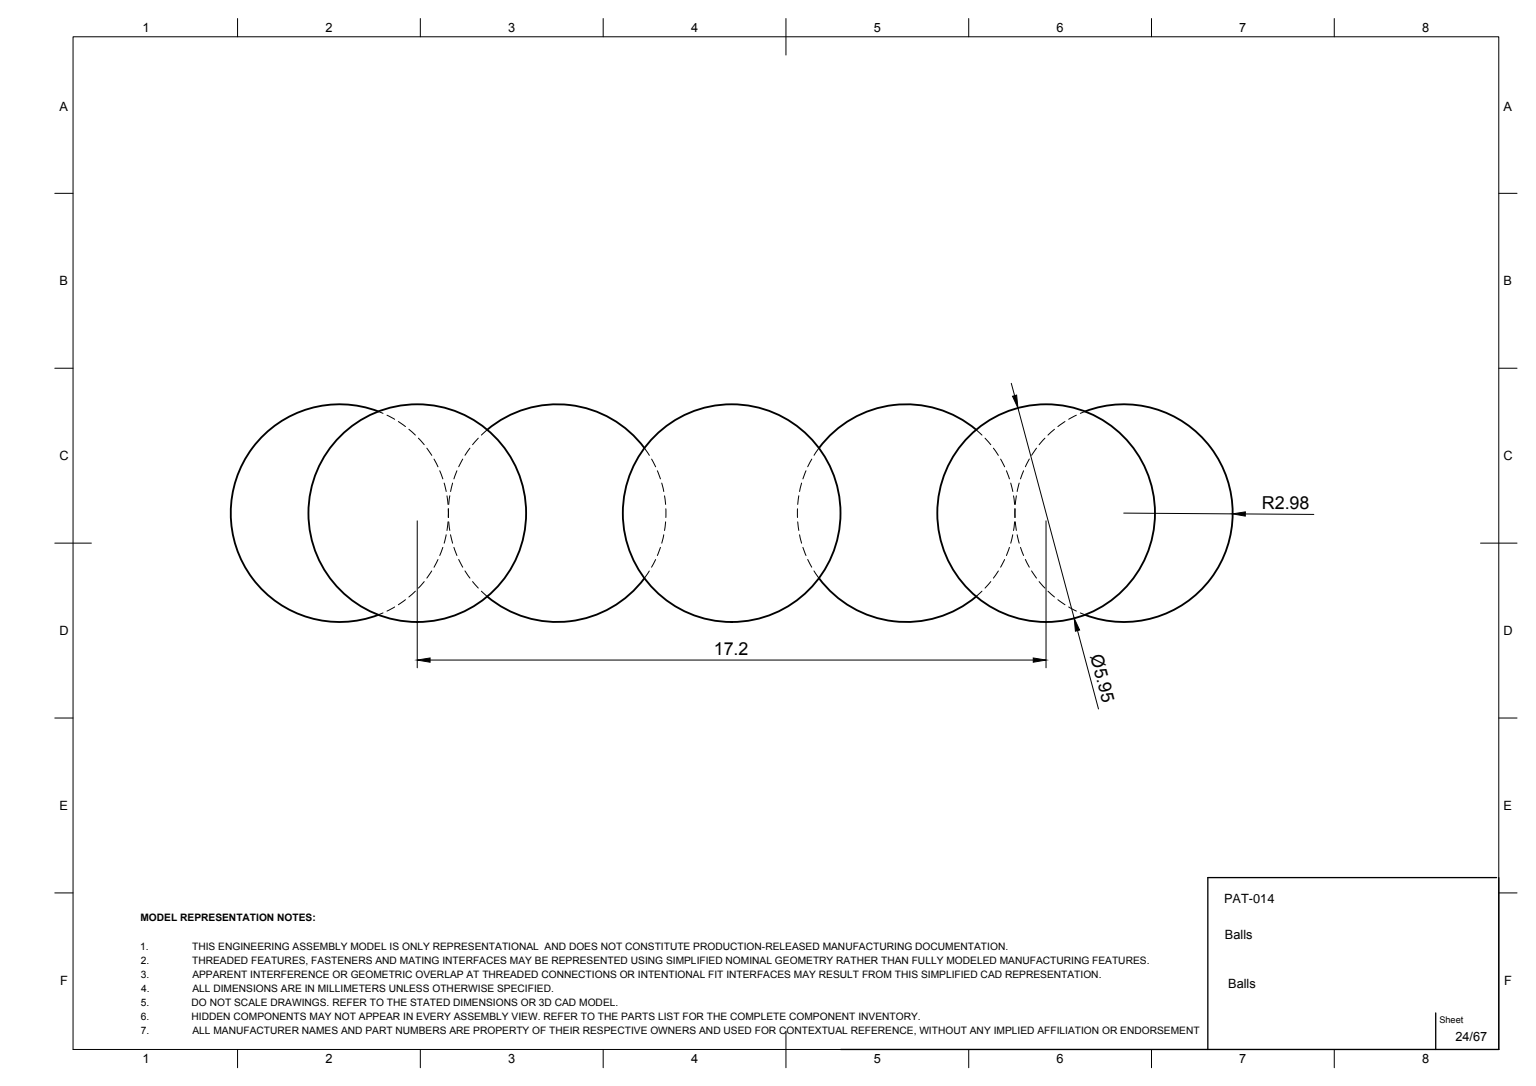
ISO-10303-21;
HEADER;
/* Generated by software containing ST-Developer
 * from STEP Tools, Inc. (www.steptools.com) 
 */

FILE_DESCRIPTION(
/* description */ ('Bin tilter linkage'),
/* implementation_level */ '2;1');

FILE_NAME(
/* name */ 'Balls.step',
/* time_stamp */ '2026-10-28T03:26:24-07:00',
/* author */ (''),
/* organization */ (''),
/* preprocessor_version */ 'ST-DEVELOPER v20.2',
/* originating_system */ 'Autodesk Translation Framework v15.17.0.0',
/* authorisation */ '');

FILE_SCHEMA (('AUTOMOTIVE_DESIGN { 1 0 10303 214 3 1 1 }'));
ENDSEC;

DATA;
#10=MECHANICAL_DESIGN_GEOMETRIC_PRESENTATION_REPRESENTATION('',(#936,#937,#938,#939,#940,#941,#942),#23728);
#613=SPHERICAL_SURFACE('',#14815,0.29765);
#614=SPHERICAL_SURFACE('',#14817,0.29765);
#615=SPHERICAL_SURFACE('',#14819,0.29765);
#616=SPHERICAL_SURFACE('',#14821,0.29765);
#617=SPHERICAL_SURFACE('',#14823,0.29765);
#618=SPHERICAL_SURFACE('',#14825,0.29765);
#619=SPHERICAL_SURFACE('',#14827,0.29765);
#724=SHAPE_REPRESENTATION_RELATIONSHIP('SRR','None',#24191,#830);
#830=ADVANCED_BREP_SHAPE_REPRESENTATION('',(#1049,#1050,#1051,#1052,#1053,
#1054,#1055),#23691);
#936=STYLED_ITEM('',(#24765),#1049);
#937=STYLED_ITEM('',(#24765),#1050);
#938=STYLED_ITEM('',(#24765),#1051);
#939=STYLED_ITEM('',(#24765),#1052);
#940=STYLED_ITEM('',(#24765),#1053);
#941=STYLED_ITEM('',(#24765),#1054);
#942=STYLED_ITEM('',(#24765),#1055);
#1049=MANIFOLD_SOLID_BREP('Body1',#12467);
#1050=MANIFOLD_SOLID_BREP('Body2',#12468);
#1051=MANIFOLD_SOLID_BREP('Body3',#12469);
#1052=MANIFOLD_SOLID_BREP('Body4',#12470);
#1053=MANIFOLD_SOLID_BREP('Body5',#12471);
#1054=MANIFOLD_SOLID_BREP('Body6',#12472);
#1055=MANIFOLD_SOLID_BREP('Body7',#12473);
#2411=FACE_OUTER_BOUND('',#3491,.T.);
#2412=FACE_OUTER_BOUND('',#3492,.T.);
#2413=FACE_OUTER_BOUND('',#3493,.T.);
#2414=FACE_OUTER_BOUND('',#3494,.T.);
#2415=FACE_OUTER_BOUND('',#3495,.T.);
#2416=FACE_OUTER_BOUND('',#3496,.T.);
#2417=FACE_OUTER_BOUND('',#3497,.T.);
#3491=EDGE_LOOP('',(#10277,#10278));
#3492=EDGE_LOOP('',(#10279,#10280));
#3493=EDGE_LOOP('',(#10281,#10282));
#3494=EDGE_LOOP('',(#10283,#10284));
#3495=EDGE_LOOP('',(#10285,#10286));
#3496=EDGE_LOOP('',(#10287,#10288));
#3497=EDGE_LOOP('',(#10289,#10290));
#5737=CIRCLE('',#14816,0.29765);
#5738=CIRCLE('',#14818,0.29765);
#5739=CIRCLE('',#14820,0.29765);
#5740=CIRCLE('',#14822,0.29765);
#5741=CIRCLE('',#14824,0.29765);
#5742=CIRCLE('',#14826,0.29765);
#5743=CIRCLE('',#14828,0.29765);
#6589=VERTEX_POINT('',#21931);
#6590=VERTEX_POINT('',#21932);
#6591=VERTEX_POINT('',#21935);
#6592=VERTEX_POINT('',#21936);
#6593=VERTEX_POINT('',#21939);
#6594=VERTEX_POINT('',#21940);
#6595=VERTEX_POINT('',#21943);
#6596=VERTEX_POINT('',#21944);
#6597=VERTEX_POINT('',#21947);
#6598=VERTEX_POINT('',#21948);
#6599=VERTEX_POINT('',#21951);
#6600=VERTEX_POINT('',#21952);
#6601=VERTEX_POINT('',#21955);
#6602=VERTEX_POINT('',#21956);
#7878=EDGE_CURVE('',#6589,#6590,#5737,.T.);
#7879=EDGE_CURVE('',#6591,#6592,#5738,.T.);
#7880=EDGE_CURVE('',#6593,#6594,#5739,.T.);
#7881=EDGE_CURVE('',#6595,#6596,#5740,.T.);
#7882=EDGE_CURVE('',#6597,#6598,#5741,.T.);
#7883=EDGE_CURVE('',#6599,#6600,#5742,.T.);
#7884=EDGE_CURVE('',#6601,#6602,#5743,.T.);
#10277=ORIENTED_EDGE('',*,*,#7878,.T.);
#10278=ORIENTED_EDGE('',*,*,#7878,.F.);
#10279=ORIENTED_EDGE('',*,*,#7879,.T.);
#10280=ORIENTED_EDGE('',*,*,#7879,.F.);
#10281=ORIENTED_EDGE('',*,*,#7880,.T.);
#10282=ORIENTED_EDGE('',*,*,#7880,.F.);
#10283=ORIENTED_EDGE('',*,*,#7881,.T.);
#10284=ORIENTED_EDGE('',*,*,#7881,.F.);
#10285=ORIENTED_EDGE('',*,*,#7882,.T.);
#10286=ORIENTED_EDGE('',*,*,#7882,.F.);
#10287=ORIENTED_EDGE('',*,*,#7883,.T.);
#10288=ORIENTED_EDGE('',*,*,#7883,.F.);
#10289=ORIENTED_EDGE('',*,*,#7884,.T.);
#10290=ORIENTED_EDGE('',*,*,#7884,.F.);
#12136=ADVANCED_FACE('',(#2411),#613,.T.);
#12137=ADVANCED_FACE('',(#2412),#614,.T.);
#12138=ADVANCED_FACE('',(#2413),#615,.T.);
#12139=ADVANCED_FACE('',(#2414),#616,.T.);
#12140=ADVANCED_FACE('',(#2415),#617,.T.);
#12141=ADVANCED_FACE('',(#2416),#618,.T.);
#12142=ADVANCED_FACE('',(#2417),#619,.T.);
#12467=CLOSED_SHELL('',(#12136));
#12468=CLOSED_SHELL('',(#12137));
#12469=CLOSED_SHELL('',(#12138));
#12470=CLOSED_SHELL('',(#12139));
#12471=CLOSED_SHELL('',(#12140));
#12472=CLOSED_SHELL('',(#12141));
#12473=CLOSED_SHELL('',(#12142));
#14814=AXIS2_PLACEMENT_3D('',#21929,#18164,#18165);
#14815=AXIS2_PLACEMENT_3D('',#21930,#18166,#18167);
#14816=AXIS2_PLACEMENT_3D('',#21933,#18168,#18169);
#14817=AXIS2_PLACEMENT_3D('',#21934,#18170,#18171);
#14818=AXIS2_PLACEMENT_3D('',#21937,#18172,#18173);
#14819=AXIS2_PLACEMENT_3D('',#21938,#18174,#18175);
#14820=AXIS2_PLACEMENT_3D('',#21941,#18176,#18177);
#14821=AXIS2_PLACEMENT_3D('',#21942,#18178,#18179);
#14822=AXIS2_PLACEMENT_3D('',#21945,#18180,#18181);
#14823=AXIS2_PLACEMENT_3D('',#21946,#18182,#18183);
#14824=AXIS2_PLACEMENT_3D('',#21949,#18184,#18185);
#14825=AXIS2_PLACEMENT_3D('',#21950,#18186,#18187);
#14826=AXIS2_PLACEMENT_3D('',#21953,#18188,#18189);
#14827=AXIS2_PLACEMENT_3D('',#21954,#18190,#18191);
#14828=AXIS2_PLACEMENT_3D('',#21957,#18192,#18193);
#18164=DIRECTION('axis',(0.,0.,1.));
#18165=DIRECTION('refdir',(1.,0.,0.));
#18166=DIRECTION('center_axis',(0.,0.,1.));
#18167=DIRECTION('ref_axis',(1.,0.,0.));
#18168=DIRECTION('center_axis',(1.22464679914735E-16,-1.,0.));
#18169=DIRECTION('ref_axis',(-1.,-1.22464679914735E-16,0.));
#18170=DIRECTION('center_axis',(0.78183148246803,0.,0.623489801858733));
#18171=DIRECTION('ref_axis',(0.623489801858734,0.,-0.78183148246803));
#18172=DIRECTION('center_axis',(7.63554790147315E-17,-1.,-9.57467422477103E-17));
#18173=DIRECTION('ref_axis',(-0.623489801858734,-1.22464679914735E-16,0.78183148246803));
#18174=DIRECTION('center_axis',(0.974927912181824,0.,-0.222520933956314));
#18175=DIRECTION('ref_axis',(-0.222520933956314,0.,-0.974927912181824));
#18176=DIRECTION('center_axis',(-2.7250954951288E-17,-1.,-1.19394234705288E-16));
#18177=DIRECTION('ref_axis',(0.222520933956314,-1.22464679914735E-16,0.974927912181824));
#18178=DIRECTION('center_axis',(0.433883739117558,0.,-0.900968867902419));
#18179=DIRECTION('ref_axis',(-0.900968867902419,0.,-0.433883739117558));
#18180=DIRECTION('center_axis',(-1.10336864020811E-16,-1.,-5.31354332312403E-17));
#18181=DIRECTION('ref_axis',(0.900968867902419,-1.22464679914735E-16,0.433883739117558));
#18182=DIRECTION('center_axis',(-0.433883739117558,0.,-0.900968867902419));
#18183=DIRECTION('ref_axis',(-0.900968867902419,0.,0.433883739117558));
#18184=DIRECTION('center_axis',(-1.10336864020811E-16,-1.,5.31354332312403E-17));
#18185=DIRECTION('ref_axis',(0.900968867902419,-1.22464679914735E-16,-0.433883739117558));
#18186=DIRECTION('center_axis',(-0.974927912181824,0.,-0.222520933956314));
#18187=DIRECTION('ref_axis',(-0.222520933956315,0.,0.974927912181824));
#18188=DIRECTION('center_axis',(-2.7250954951288E-17,-1.,1.19394234705288E-16));
#18189=DIRECTION('ref_axis',(0.222520933956315,-1.22464679914735E-16,-0.974927912181824));
#18190=DIRECTION('center_axis',(-0.78183148246803,0.,0.623489801858734));
#18191=DIRECTION('ref_axis',(0.623489801858733,0.,0.78183148246803));
#18192=DIRECTION('center_axis',(7.63554790147315E-17,-1.,9.57467422477103E-17));
#18193=DIRECTION('ref_axis',(-0.623489801858733,-1.22464679914735E-16,-0.78183148246803));
#21929=CARTESIAN_POINT('',(0.,0.,0.));
#21930=CARTESIAN_POINT('Origin',(1.1,0.,0.));
#21931=CARTESIAN_POINT('',(1.1,-2.23201749654651E-33,0.29765));
#21932=CARTESIAN_POINT('',(1.1,-2.23201749654651E-33,-0.29765));
#21933=CARTESIAN_POINT('Origin',(1.1,0.,0.));
#21934=CARTESIAN_POINT('Origin',(0.685838782044607,0.,-0.860014630714833));
#21935=CARTESIAN_POINT('',(0.918550922801216,-5.31350540756609E-33,-0.674432891191581));
#21936=CARTESIAN_POINT('',(0.453126641287998,8.49470414473068E-34,-1.04559637023808));
#21937=CARTESIAN_POINT('Origin',(0.685838782044607,0.,-0.860014630714833));
#21938=CARTESIAN_POINT('Origin',(-0.244773027351946,0.,-1.07242070340001));
#21939=CARTESIAN_POINT('',(0.0454142657089739,-2.23201749654651E-33,-1.1386540593921));
#21940=CARTESIAN_POINT('',(-0.534960320412865,-2.23201749654651E-33,-1.00618734740791));
#21941=CARTESIAN_POINT('Origin',(-0.244773027351946,0.,-1.07242070340001));
#21942=CARTESIAN_POINT('Origin',(-0.991065754692661,0.,-0.477272113029314));
#21943=CARTESIAN_POINT('',(-0.86192025974432,8.49470414473067E-34,-0.745445496560469));
#21944=CARTESIAN_POINT('',(-1.120211249641,-5.31350540756609E-33,-0.209098729498159));
#21945=CARTESIAN_POINT('Origin',(-0.991065754692661,0.,-0.477272113029314));
#21946=CARTESIAN_POINT('Origin',(-0.991065754692661,0.,0.477272113029314));
#21947=CARTESIAN_POINT('',(-1.120211249641,-2.23201749654651E-33,0.209098729498159));
#21948=CARTESIAN_POINT('',(-0.86192025974432,-2.23201749654651E-33,0.745445496560469));
#21949=CARTESIAN_POINT('Origin',(-0.991065754692661,0.,0.477272113029314));
#21950=CARTESIAN_POINT('Origin',(-0.244773027351946,0.,1.07242070340001));
#21951=CARTESIAN_POINT('',(-0.534960320412866,-2.23201749654651E-33,1.00618734740791));
#21952=CARTESIAN_POINT('',(0.0454142657089737,-2.23201749654651E-33,1.1386540593921));
#21953=CARTESIAN_POINT('Origin',(-0.244773027351946,0.,1.07242070340001));
#21954=CARTESIAN_POINT('Origin',(0.685838782044607,0.,0.860014630714833));
#21955=CARTESIAN_POINT('',(0.453126641287998,-2.23201749654651E-33,1.04559637023808));
#21956=CARTESIAN_POINT('',(0.918550922801216,-2.23201749654651E-33,0.674432891191581));
#21957=CARTESIAN_POINT('Origin',(0.685838782044607,0.,0.860014630714833));
#23574=UNCERTAINTY_MEASURE_WITH_UNIT(LENGTH_MEASURE(0.001),#23729,
'DISTANCE_ACCURACY_VALUE',
'Maximum model space distance between geometric entities at asserted c
onnectivities');
#23611=UNCERTAINTY_MEASURE_WITH_UNIT(LENGTH_MEASURE(0.001),#23729,
'DISTANCE_ACCURACY_VALUE',
'Maximum model space distance between geometric entities at asserted c
onnectivities');
#23691=(
GEOMETRIC_REPRESENTATION_CONTEXT(3)
GLOBAL_UNCERTAINTY_ASSIGNED_CONTEXT((#23574))
GLOBAL_UNIT_ASSIGNED_CONTEXT((#23729,#23731,#23732))
REPRESENTATION_CONTEXT('','3D')
);
#23728=(
GEOMETRIC_REPRESENTATION_CONTEXT(3)
GLOBAL_UNCERTAINTY_ASSIGNED_CONTEXT((#23611))
GLOBAL_UNIT_ASSIGNED_CONTEXT((#23729,#23731,#23732))
REPRESENTATION_CONTEXT('','3D')
);
#23729=(
LENGTH_UNIT()
NAMED_UNIT(*)
SI_UNIT(.CENTI.,.METRE.)
);
#23731=(
NAMED_UNIT(*)
PLANE_ANGLE_UNIT()
SI_UNIT($,.RADIAN.)
);
#23732=(
NAMED_UNIT(*)
SI_UNIT($,.STERADIAN.)
SOLID_ANGLE_UNIT()
);
#23812=SHAPE_DEFINITION_REPRESENTATION(#23928,#24191);
#23928=PRODUCT_DEFINITION_SHAPE('',$,#24308);
#24191=SHAPE_REPRESENTATION('',(#14814),#23691);
#24228=PRODUCT_DEFINITION_CONTEXT('part definition',#24578,'design');
#24308=PRODUCT_DEFINITION('Balls','Balls',#24424,#24228);
#24424=PRODUCT_DEFINITION_FORMATION('',$,#24659);
#24578=APPLICATION_CONTEXT(
'Core Data for Automotive Mechanical Design Process');
#24579=PRODUCT_CONTEXT('part definition',#24578,'mechanical');
#24659=PRODUCT('Balls','Balls','Balls',(#24579));
#24759=COLOUR_RGB('Grey',0.48,0.52,0.57);
#24760=FILL_AREA_STYLE_COLOUR('',#24759);
#24761=FILL_AREA_STYLE('',(#24760));
#24762=SURFACE_STYLE_FILL_AREA(#24761);
#24763=SURFACE_SIDE_STYLE('',(#24762));
#24764=SURFACE_STYLE_USAGE(.BOTH.,#24763);
#24765=PRESENTATION_STYLE_ASSIGNMENT((#24764));
ENDSEC;
END-ISO-10303-21;
